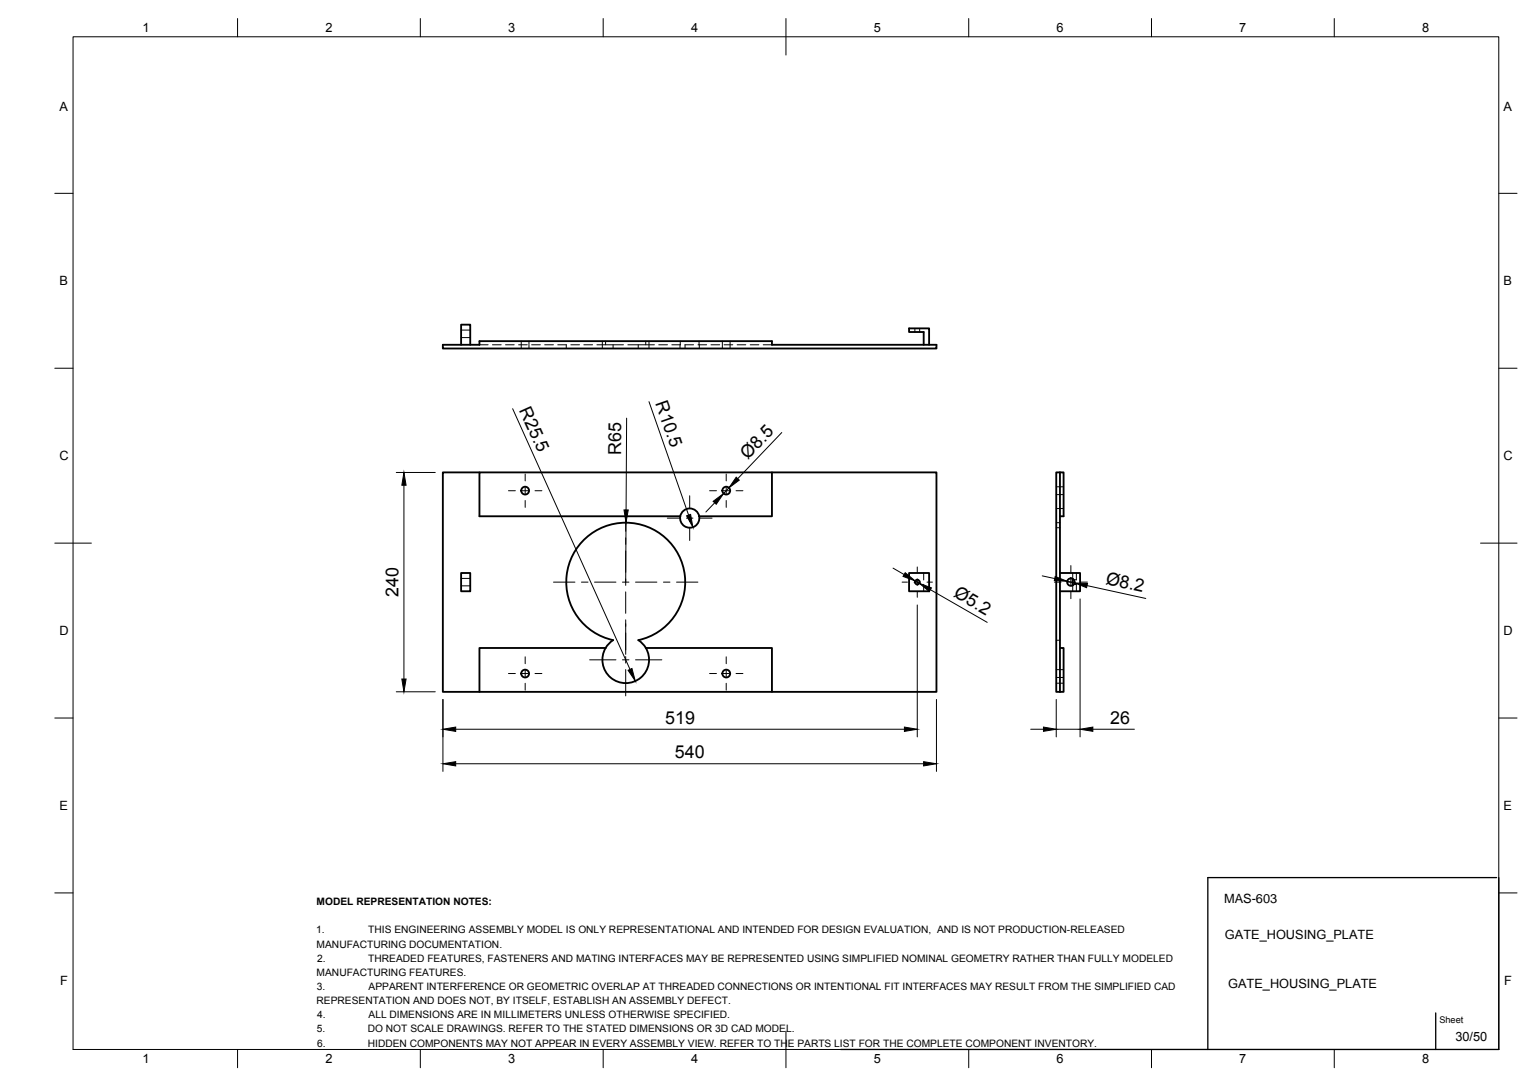
ISO-10303-21;
HEADER;
FILE_DESCRIPTION((''),'2;1');
FILE_NAME('GATE_HOUSING_PLATE.step','2026-10-01T22:06:14-07:00',(''),(''),'','','');
FILE_SCHEMA (('AUTOMOTIVE_DESIGN { 1 0 10303 214 3 1 1 }'));
ENDSEC;
DATA;
#10=MECHANICAL_DESIGN_GEOMETRIC_PRESENTATION_REPRESENTATION('',(#1002),#50440);
#910=SHAPE_REPRESENTATION_RELATIONSHIP('SRR','None',#50643,#955) ;
#955=ADVANCED_BREP_SHAPE_REPRESENTATION('',(#1057),#50412) ;
#1002=STYLED_ITEM('',(#50885),#1057) ;
#1057=MANIFOLD_SOLID_BREP('GATE_HOUSING_PLATE',#28669) ;
#1316=FACE_BOUND('',#5009,.T.) ;
#1317=FACE_BOUND('',#5014,.T.) ;
#1318=FACE_BOUND('',#5021,.T.) ;
#1319=FACE_BOUND('',#5024,.T.) ;
#1320=FACE_BOUND('',#5031,.T.) ;
#1321=FACE_BOUND('',#5032,.T.) ;
#1322=FACE_BOUND('',#5035,.T.) ;
#1323=FACE_BOUND('',#5036,.T.) ;
#1324=FACE_BOUND('',#5042,.T.) ;
#1325=FACE_BOUND('',#5043,.T.) ;
#1326=FACE_BOUND('',#5049,.T.) ;
#1327=FACE_BOUND('',#5050,.T.) ;
#1328=FACE_BOUND('',#5051,.T.) ;
#1329=FACE_BOUND('',#5052,.T.) ;
#1330=FACE_BOUND('',#5053,.T.) ;
#1331=FACE_BOUND('',#5054,.T.) ;
#2103=PLANE('',#30678) ;
#2104=PLANE('',#30679) ;
#2105=PLANE('',#30680) ;
#2106=PLANE('',#30681) ;
#2107=PLANE('',#30682) ;
#2108=PLANE('',#30683) ;
#2109=PLANE('',#30684) ;
#2110=PLANE('',#30688) ;
#2111=PLANE('',#30689) ;
#2112=PLANE('',#30690) ;
#2113=PLANE('',#30691) ;
#2114=PLANE('',#30692) ;
#2115=PLANE('',#30710) ;
#2116=PLANE('',#30714) ;
#2117=PLANE('',#30715) ;
#2118=PLANE('',#30717) ;
#2119=PLANE('',#30718) ;
#2120=PLANE('',#30719) ;
#2121=PLANE('',#30720) ;
#2122=PLANE('',#30721) ;
#2123=PLANE('',#30722) ;
#2124=PLANE('',#30723) ;
#2125=PLANE('',#30724) ;
#2126=PLANE('',#30727) ;
#2127=PLANE('',#30730) ;
#2128=PLANE('',#30731) ;
#2129=PLANE('',#30732) ;
#2130=PLANE('',#30733) ;
#3249=FACE_OUTER_BOUND('',#5007,.T.) ;
#3250=FACE_OUTER_BOUND('',#5008,.T.) ;
#3251=FACE_OUTER_BOUND('',#5010,.T.) ;
#3252=FACE_OUTER_BOUND('',#5011,.T.) ;
#3253=FACE_OUTER_BOUND('',#5012,.T.) ;
#3254=FACE_OUTER_BOUND('',#5013,.T.) ;
#3255=FACE_OUTER_BOUND('',#5015,.T.) ;
#3256=FACE_OUTER_BOUND('',#5016,.T.) ;
#3257=FACE_OUTER_BOUND('',#5017,.T.) ;
#3258=FACE_OUTER_BOUND('',#5018,.T.) ;
#3259=FACE_OUTER_BOUND('',#5019,.T.) ;
#3260=FACE_OUTER_BOUND('',#5020,.T.) ;
#3261=FACE_OUTER_BOUND('',#5022,.T.) ;
#3262=FACE_OUTER_BOUND('',#5023,.T.) ;
#3263=FACE_OUTER_BOUND('',#5025,.T.) ;
#3264=FACE_OUTER_BOUND('',#5026,.T.) ;
#3265=FACE_OUTER_BOUND('',#5027,.T.) ;
#3266=FACE_OUTER_BOUND('',#5028,.T.) ;
#3267=FACE_OUTER_BOUND('',#5029,.T.) ;
#3268=FACE_OUTER_BOUND('',#5030,.T.) ;
#3269=FACE_OUTER_BOUND('',#5033,.T.) ;
#3270=FACE_OUTER_BOUND('',#5034,.T.) ;
#3271=FACE_OUTER_BOUND('',#5037,.T.) ;
#3272=FACE_OUTER_BOUND('',#5038,.T.) ;
#3273=FACE_OUTER_BOUND('',#5039,.T.) ;
#3274=FACE_OUTER_BOUND('',#5040,.T.) ;
#3275=FACE_OUTER_BOUND('',#5041,.T.) ;
#3276=FACE_OUTER_BOUND('',#5044,.T.) ;
#3277=FACE_OUTER_BOUND('',#5045,.T.) ;
#3278=FACE_OUTER_BOUND('',#5046,.T.) ;
#3279=FACE_OUTER_BOUND('',#5047,.T.) ;
#3280=FACE_OUTER_BOUND('',#5048,.T.) ;
#3281=FACE_OUTER_BOUND('',#5055,.T.) ;
#3282=FACE_OUTER_BOUND('',#5056,.T.) ;
#3283=FACE_OUTER_BOUND('',#5057,.T.) ;
#3284=FACE_OUTER_BOUND('',#5058,.T.) ;
#3285=FACE_OUTER_BOUND('',#5059,.T.) ;
#5007=EDGE_LOOP('',(#23237,#23238,#23239,#23240)) ;
#5008=EDGE_LOOP('',(#23241,#23242,#23243,#23244)) ;
#5009=EDGE_LOOP('',(#23245)) ;
#5010=EDGE_LOOP('',(#23246,#23247,#23248,#23249)) ;
#5011=EDGE_LOOP('',(#23250,#23251,#23252,#23253,#23254,#23255)) ;
#5012=EDGE_LOOP('',(#23256,#23257,#23258,#23259)) ;
#5013=EDGE_LOOP('',(#23260,#23261,#23262,#23263)) ;
#5014=EDGE_LOOP('',(#23264)) ;
#5015=EDGE_LOOP('',(#23265,#23266,#23267,#23268,#23269,#23270)) ;
#5016=EDGE_LOOP('',(#23271,#23272,#23273,#23274)) ;
#5017=EDGE_LOOP('',(#23275,#23276,#23277,#23278)) ;
#5018=EDGE_LOOP('',(#23279,#23280,#23281,#23282)) ;
#5019=EDGE_LOOP('',(#23283,#23284,#23285,#23286)) ;
#5020=EDGE_LOOP('',(#23287,#23288,#23289,#23290)) ;
#5021=EDGE_LOOP('',(#23291)) ;
#5022=EDGE_LOOP('',(#23292,#23293,#23294,#23295)) ;
#5023=EDGE_LOOP('',(#23296,#23297,#23298,#23299)) ;
#5024=EDGE_LOOP('',(#23300)) ;
#5025=EDGE_LOOP('',(#23301,#23302,#23303,#23304)) ;
#5026=EDGE_LOOP('',(#23305,#23306,#23307,#23308)) ;
#5027=EDGE_LOOP('',(#23309,#23310,#23311,#23312)) ;
#5028=EDGE_LOOP('',(#23313,#23314,#23315,#23316)) ;
#5029=EDGE_LOOP('',(#23317,#23318,#23319,#23320,#23321,#23322,#23323,#23324)) ;
#5030=EDGE_LOOP('',(#23325,#23326,#23327,#23328,#23329,#23330,#23331,#23332,
#23333,#23334,#23335,#23336,#23337,#23338,#23339,#23340,#23341,#23342,#23343)) ;
#5031=EDGE_LOOP('',(#23344,#23345,#23346,#23347)) ;
#5032=EDGE_LOOP('',(#23348,#23349,#23350,#23351)) ;
#5033=EDGE_LOOP('',(#23352,#23353,#23354,#23355)) ;
#5034=EDGE_LOOP('',(#23356,#23357,#23358,#23359,#23360,#23361)) ;
#5035=EDGE_LOOP('',(#23362)) ;
#5036=EDGE_LOOP('',(#23363)) ;
#5037=EDGE_LOOP('',(#23364,#23365,#23366,#23367)) ;
#5038=EDGE_LOOP('',(#23368,#23369,#23370,#23371)) ;
#5039=EDGE_LOOP('',(#23372,#23373,#23374,#23375)) ;
#5040=EDGE_LOOP('',(#23376,#23377,#23378,#23379)) ;
#5041=EDGE_LOOP('',(#23380,#23381,#23382,#23383,#23384,#23385)) ;
#5042=EDGE_LOOP('',(#23386)) ;
#5043=EDGE_LOOP('',(#23387)) ;
#5044=EDGE_LOOP('',(#23388,#23389,#23390,#23391)) ;
#5045=EDGE_LOOP('',(#23392,#23393,#23394,#23395)) ;
#5046=EDGE_LOOP('',(#23396,#23397,#23398,#23399)) ;
#5047=EDGE_LOOP('',(#23400,#23401,#23402,#23403,#23404,#23405,#23406,#23407)) ;
#5048=EDGE_LOOP('',(#23408,#23409,#23410,#23411)) ;
#5049=EDGE_LOOP('',(#23412)) ;
#5050=EDGE_LOOP('',(#23413)) ;
#5051=EDGE_LOOP('',(#23414)) ;
#5052=EDGE_LOOP('',(#23415)) ;
#5053=EDGE_LOOP('',(#23416)) ;
#5054=EDGE_LOOP('',(#23417,#23418)) ;
#5055=EDGE_LOOP('',(#23419,#23420,#23421,#23422)) ;
#5056=EDGE_LOOP('',(#23423,#23424,#23425,#23426,#23427,#23428,#23429,#23430)) ;
#5057=EDGE_LOOP('',(#23431,#23432,#23433,#23434)) ;
#5058=EDGE_LOOP('',(#23435,#23436,#23437,#23438,#23439,#23440,#23441,#23442)) ;
#5059=EDGE_LOOP('',(#23443,#23444,#23445,#23446)) ;
#7537=LINE('',#46216,#10009) ;
#7538=LINE('',#46221,#10010) ;
#7539=LINE('',#46223,#10011) ;
#7540=LINE('',#46225,#10012) ;
#7541=LINE('',#46226,#10013) ;
#7542=LINE('',#46229,#10014) ;
#7543=LINE('',#46231,#10015) ;
#7544=LINE('',#46232,#10016) ;
#7545=LINE('',#46236,#10017) ;
#7546=LINE('',#46238,#10018) ;
#7547=LINE('',#46239,#10019) ;
#7548=LINE('',#46240,#10020) ;
#7549=LINE('',#46244,#10021) ;
#7550=LINE('',#46245,#10022) ;
#7551=LINE('',#46246,#10023) ;
#7552=LINE('',#46248,#10024) ;
#7553=LINE('',#46251,#10025) ;
#7554=LINE('',#46252,#10026) ;
#7555=LINE('',#46254,#10027) ;
#7556=LINE('',#46259,#10028) ;
#7557=LINE('',#46264,#10029) ;
#7558=LINE('',#46266,#10030) ;
#7559=LINE('',#46268,#10031) ;
#7560=LINE('',#46269,#10032) ;
#7561=LINE('',#46272,#10033) ;
#7562=LINE('',#46274,#10034) ;
#7563=LINE('',#46275,#10035) ;
#7564=LINE('',#46278,#10036) ;
#7565=LINE('',#46279,#10037) ;
#7566=LINE('',#46282,#10038) ;
#7567=LINE('',#46283,#10039) ;
#7568=LINE('',#46285,#10040) ;
#7569=LINE('',#46290,#10041) ;
#7570=LINE('',#46296,#10042) ;
#7571=LINE('',#46302,#10043) ;
#7572=LINE('',#46308,#10044) ;
#7573=LINE('',#46314,#10045) ;
#7574=LINE('',#46318,#10046) ;
#7575=LINE('',#46322,#10047) ;
#7576=LINE('',#46326,#10048) ;
#7577=LINE('',#46328,#10049) ;
#7578=LINE('',#46330,#10050) ;
#7579=LINE('',#46332,#10051) ;
#7580=LINE('',#46334,#10052) ;
#7581=LINE('',#46336,#10053) ;
#7582=LINE('',#46338,#10054) ;
#7583=LINE('',#46346,#10055) ;
#7584=LINE('',#46348,#10056) ;
#7585=LINE('',#46350,#10057) ;
#7586=LINE('',#46352,#10058) ;
#7587=LINE('',#46354,#10059) ;
#7588=LINE('',#46356,#10060) ;
#7589=LINE('',#46357,#10061) ;
#7590=LINE('',#46360,#10062) ;
#7591=LINE('',#46361,#10063) ;
#7592=LINE('',#46367,#10064) ;
#7593=LINE('',#46369,#10065) ;
#7594=LINE('',#46371,#10066) ;
#7595=LINE('',#46373,#10067) ;
#7596=LINE('',#46374,#10068) ;
#7597=LINE('',#46376,#10069) ;
#7598=LINE('',#46377,#10070) ;
#7599=LINE('',#46379,#10071) ;
#7600=LINE('',#46381,#10072) ;
#7601=LINE('',#46382,#10073) ;
#7602=LINE('',#46384,#10074) ;
#7603=LINE('',#46387,#10075) ;
#7604=LINE('',#46389,#10076) ;
#7605=LINE('',#46391,#10077) ;
#7606=LINE('',#46392,#10078) ;
#7607=LINE('',#46394,#10079) ;
#7608=LINE('',#46396,#10080) ;
#7609=LINE('',#46398,#10081) ;
#7610=LINE('',#46401,#10082) ;
#7611=LINE('',#46404,#10083) ;
#7612=LINE('',#46408,#10084) ;
#7613=LINE('',#46410,#10085) ;
#7614=LINE('',#46412,#10086) ;
#7615=LINE('',#46413,#10087) ;
#7616=LINE('',#46417,#10088) ;
#7617=LINE('',#46418,#10089) ;
#7618=LINE('',#46420,#10090) ;
#7619=LINE('',#46422,#10091) ;
#10009=VECTOR('',#37116,0.26) ;
#10010=VECTOR('',#37121,1.) ;
#10011=VECTOR('',#37122,1.) ;
#10012=VECTOR('',#37123,1.) ;
#10013=VECTOR('',#37124,1.) ;
#10014=VECTOR('',#37127,1.) ;
#10015=VECTOR('',#37128,1.) ;
#10016=VECTOR('',#37129,1.) ;
#10017=VECTOR('',#37132,1.) ;
#10018=VECTOR('',#37133,1.) ;
#10019=VECTOR('',#37134,1.) ;
#10020=VECTOR('',#37135,1.) ;
#10021=VECTOR('',#37138,1.) ;
#10022=VECTOR('',#37139,1.) ;
#10023=VECTOR('',#37140,1.) ;
#10024=VECTOR('',#37143,1.) ;
#10025=VECTOR('',#37146,1.) ;
#10026=VECTOR('',#37147,1.) ;
#10027=VECTOR('',#37150,1.) ;
#10028=VECTOR('',#37155,0.41) ;
#10029=VECTOR('',#37160,1.) ;
#10030=VECTOR('',#37161,1.) ;
#10031=VECTOR('',#37162,1.) ;
#10032=VECTOR('',#37163,1.) ;
#10033=VECTOR('',#37166,1.) ;
#10034=VECTOR('',#37167,1.) ;
#10035=VECTOR('',#37168,1.) ;
#10036=VECTOR('',#37171,1.) ;
#10037=VECTOR('',#37172,1.) ;
#10038=VECTOR('',#37175,1.) ;
#10039=VECTOR('',#37176,1.) ;
#10040=VECTOR('',#37179,1.) ;
#10041=VECTOR('',#37184,0.425) ;
#10042=VECTOR('',#37191,0.425) ;
#10043=VECTOR('',#37198,0.425) ;
#10044=VECTOR('',#37205,0.425) ;
#10045=VECTOR('',#37212,1.05) ;
#10046=VECTOR('',#37215,1.) ;
#10047=VECTOR('',#37218,1.) ;
#10048=VECTOR('',#37223,1.) ;
#10049=VECTOR('',#37224,1.) ;
#10050=VECTOR('',#37225,1.) ;
#10051=VECTOR('',#37226,1.) ;
#10052=VECTOR('',#37227,1.) ;
#10053=VECTOR('',#37228,1.) ;
#10054=VECTOR('',#37229,1.) ;
#10055=VECTOR('',#37236,1.) ;
#10056=VECTOR('',#37237,1.) ;
#10057=VECTOR('',#37238,1.) ;
#10058=VECTOR('',#37239,1.) ;
#10059=VECTOR('',#37240,1.) ;
#10060=VECTOR('',#37241,1.) ;
#10061=VECTOR('',#37242,1.) ;
#10062=VECTOR('',#37245,1.) ;
#10063=VECTOR('',#37246,1.) ;
#10064=VECTOR('',#37251,1.) ;
#10065=VECTOR('',#37252,1.) ;
#10066=VECTOR('',#37253,1.) ;
#10067=VECTOR('',#37254,1.) ;
#10068=VECTOR('',#37255,1.) ;
#10069=VECTOR('',#37258,1.) ;
#10070=VECTOR('',#37259,1.) ;
#10071=VECTOR('',#37262,1.) ;
#10072=VECTOR('',#37265,1.) ;
#10073=VECTOR('',#37266,1.) ;
#10074=VECTOR('',#37269,1.) ;
#10075=VECTOR('',#37272,1.) ;
#10076=VECTOR('',#37273,1.) ;
#10077=VECTOR('',#37274,1.) ;
#10078=VECTOR('',#37275,1.) ;
#10079=VECTOR('',#37278,1.) ;
#10080=VECTOR('',#37281,1.) ;
#10081=VECTOR('',#37284,1.) ;
#10082=VECTOR('',#37287,1.) ;
#10083=VECTOR('',#37290,1.) ;
#10084=VECTOR('',#37293,1.) ;
#10085=VECTOR('',#37294,1.) ;
#10086=VECTOR('',#37295,1.) ;
#10087=VECTOR('',#37296,1.) ;
#10088=VECTOR('',#37303,1.) ;
#10089=VECTOR('',#37304,1.) ;
#10090=VECTOR('',#37307,1.) ;
#10091=VECTOR('',#37310,1.) ;
#11151=CIRCLE('',#30676,0.26) ;
#11152=CIRCLE('',#30677,0.26) ;
#11153=CIRCLE('',#30686,0.41) ;
#11154=CIRCLE('',#30687,0.41) ;
#11155=CIRCLE('',#30694,0.425) ;
#11156=CIRCLE('',#30695,0.425) ;
#11157=CIRCLE('',#30697,0.425) ;
#11158=CIRCLE('',#30698,0.425) ;
#11159=CIRCLE('',#30700,0.425) ;
#11160=CIRCLE('',#30701,0.425) ;
#11161=CIRCLE('',#30703,0.425) ;
#11162=CIRCLE('',#30704,0.425) ;
#11163=CIRCLE('',#30706,1.05) ;
#11164=CIRCLE('',#30707,1.05) ;
#11165=CIRCLE('',#30708,1.05) ;
#11166=CIRCLE('',#30709,1.05) ;
#11167=CIRCLE('',#30711,2.55) ;
#11168=CIRCLE('',#30712,6.5) ;
#11169=CIRCLE('',#30713,2.55) ;
#11170=CIRCLE('',#30716,2.55) ;
#11171=CIRCLE('',#30726,2.55) ;
#11172=CIRCLE('',#30728,6.5) ;
#13395=VERTEX_POINT('',#46213) ;
#13396=VERTEX_POINT('',#46215) ;
#13397=VERTEX_POINT('',#46219) ;
#13398=VERTEX_POINT('',#46220) ;
#13399=VERTEX_POINT('',#46222) ;
#13400=VERTEX_POINT('',#46224) ;
#13401=VERTEX_POINT('',#46228) ;
#13402=VERTEX_POINT('',#46230) ;
#13403=VERTEX_POINT('',#46234) ;
#13404=VERTEX_POINT('',#46235) ;
#13405=VERTEX_POINT('',#46237) ;
#13406=VERTEX_POINT('',#46242) ;
#13407=VERTEX_POINT('',#46243) ;
#13408=VERTEX_POINT('',#46250) ;
#13409=VERTEX_POINT('',#46256) ;
#13410=VERTEX_POINT('',#46258) ;
#13411=VERTEX_POINT('',#46262) ;
#13412=VERTEX_POINT('',#46263) ;
#13413=VERTEX_POINT('',#46265) ;
#13414=VERTEX_POINT('',#46267) ;
#13415=VERTEX_POINT('',#46271) ;
#13416=VERTEX_POINT('',#46273) ;
#13417=VERTEX_POINT('',#46277) ;
#13418=VERTEX_POINT('',#46281) ;
#13419=VERTEX_POINT('',#46287) ;
#13420=VERTEX_POINT('',#46289) ;
#13421=VERTEX_POINT('',#46293) ;
#13422=VERTEX_POINT('',#46295) ;
#13423=VERTEX_POINT('',#46299) ;
#13424=VERTEX_POINT('',#46301) ;
#13425=VERTEX_POINT('',#46305) ;
#13426=VERTEX_POINT('',#46307) ;
#13427=VERTEX_POINT('',#46311) ;
#13428=VERTEX_POINT('',#46313) ;
#13429=VERTEX_POINT('',#46315) ;
#13430=VERTEX_POINT('',#46317) ;
#13431=VERTEX_POINT('',#46319) ;
#13432=VERTEX_POINT('',#46321) ;
#13433=VERTEX_POINT('',#46325) ;
#13434=VERTEX_POINT('',#46327) ;
#13435=VERTEX_POINT('',#46329) ;
#13436=VERTEX_POINT('',#46331) ;
#13437=VERTEX_POINT('',#46333) ;
#13438=VERTEX_POINT('',#46335) ;
#13439=VERTEX_POINT('',#46337) ;
#13440=VERTEX_POINT('',#46339) ;
#13441=VERTEX_POINT('',#46341) ;
#13442=VERTEX_POINT('',#46343) ;
#13443=VERTEX_POINT('',#46345) ;
#13444=VERTEX_POINT('',#46347) ;
#13445=VERTEX_POINT('',#46349) ;
#13446=VERTEX_POINT('',#46351) ;
#13447=VERTEX_POINT('',#46353) ;
#13448=VERTEX_POINT('',#46355) ;
#13449=VERTEX_POINT('',#46359) ;
#13450=VERTEX_POINT('',#46363) ;
#13451=VERTEX_POINT('',#46364) ;
#13452=VERTEX_POINT('',#46366) ;
#13453=VERTEX_POINT('',#46368) ;
#13454=VERTEX_POINT('',#46370) ;
#13455=VERTEX_POINT('',#46372) ;
#13456=VERTEX_POINT('',#46386) ;
#13457=VERTEX_POINT('',#46388) ;
#13458=VERTEX_POINT('',#46390) ;
#13459=VERTEX_POINT('',#46400) ;
#13460=VERTEX_POINT('',#46402) ;
#13461=VERTEX_POINT('',#46406) ;
#13462=VERTEX_POINT('',#46407) ;
#13463=VERTEX_POINT('',#46409) ;
#13464=VERTEX_POINT('',#46411) ;
#16884=EDGE_CURVE('',#13395,#13395,#11151,.T.) ;
#16885=EDGE_CURVE('',#13395,#13396,#7537,.T.) ;
#16886=EDGE_CURVE('',#13396,#13396,#11152,.T.) ;
#16887=EDGE_CURVE('',#13397,#13398,#7538,.T.) ;
#16888=EDGE_CURVE('',#13397,#13399,#7539,.T.) ;
#16889=EDGE_CURVE('',#13399,#13400,#7540,.T.) ;
#16890=EDGE_CURVE('',#13400,#13398,#7541,.T.) ;
#16891=EDGE_CURVE('',#13401,#13400,#7542,.T.) ;
#16892=EDGE_CURVE('',#13402,#13399,#7543,.T.) ;
#16893=EDGE_CURVE('',#13401,#13402,#7544,.T.) ;
#16894=EDGE_CURVE('',#13403,#13404,#7545,.T.) ;
#16895=EDGE_CURVE('',#13405,#13404,#7546,.T.) ;
#16896=EDGE_CURVE('',#13398,#13405,#7547,.T.) ;
#16897=EDGE_CURVE('',#13403,#13401,#7548,.T.) ;
#16898=EDGE_CURVE('',#13406,#13407,#7549,.T.) ;
#16899=EDGE_CURVE('',#13404,#13407,#7550,.T.) ;
#16900=EDGE_CURVE('',#13406,#13403,#7551,.T.) ;
#16901=EDGE_CURVE('',#13402,#13406,#7552,.T.) ;
#16902=EDGE_CURVE('',#13397,#13408,#7553,.T.) ;
#16903=EDGE_CURVE('',#13407,#13408,#7554,.T.) ;
#16904=EDGE_CURVE('',#13408,#13405,#7555,.T.) ;
#16905=EDGE_CURVE('',#13409,#13409,#11153,.T.) ;
#16906=EDGE_CURVE('',#13409,#13410,#7556,.T.) ;
#16907=EDGE_CURVE('',#13410,#13410,#11154,.T.) ;
#16908=EDGE_CURVE('',#13411,#13412,#7557,.T.) ;
#16909=EDGE_CURVE('',#13412,#13413,#7558,.T.) ;
#16910=EDGE_CURVE('',#13413,#13414,#7559,.T.) ;
#16911=EDGE_CURVE('',#13414,#13411,#7560,.T.) ;
#16912=EDGE_CURVE('',#13414,#13415,#7561,.T.) ;
#16913=EDGE_CURVE('',#13416,#13415,#7562,.T.) ;
#16914=EDGE_CURVE('',#13411,#13416,#7563,.T.) ;
#16915=EDGE_CURVE('',#13413,#13417,#7564,.T.) ;
#16916=EDGE_CURVE('',#13415,#13417,#7565,.T.) ;
#16917=EDGE_CURVE('',#13412,#13418,#7566,.T.) ;
#16918=EDGE_CURVE('',#13417,#13418,#7567,.T.) ;
#16919=EDGE_CURVE('',#13418,#13416,#7568,.T.) ;
#16920=EDGE_CURVE('',#13419,#13419,#11155,.T.) ;
#16921=EDGE_CURVE('',#13419,#13420,#7569,.T.) ;
#16922=EDGE_CURVE('',#13420,#13420,#11156,.T.) ;
#16923=EDGE_CURVE('',#13421,#13421,#11157,.T.) ;
#16924=EDGE_CURVE('',#13421,#13422,#7570,.T.) ;
#16925=EDGE_CURVE('',#13422,#13422,#11158,.T.) ;
#16926=EDGE_CURVE('',#13423,#13423,#11159,.T.) ;
#16927=EDGE_CURVE('',#13423,#13424,#7571,.T.) ;
#16928=EDGE_CURVE('',#13424,#13424,#11160,.T.) ;
#16929=EDGE_CURVE('',#13425,#13425,#11161,.T.) ;
#16930=EDGE_CURVE('',#13425,#13426,#7572,.T.) ;
#16931=EDGE_CURVE('',#13426,#13426,#11162,.T.) ;
#16932=EDGE_CURVE('',#13427,#13427,#11163,.T.) ;
#16933=EDGE_CURVE('',#13427,#13428,#7573,.T.) ;
#16934=EDGE_CURVE('',#13429,#13428,#11164,.T.) ;
#16935=EDGE_CURVE('',#13430,#13429,#7574,.T.) ;
#16936=EDGE_CURVE('',#13431,#13430,#11165,.T.) ;
#16937=EDGE_CURVE('',#13432,#13431,#7575,.T.) ;
#16938=EDGE_CURVE('',#13428,#13432,#11166,.T.) ;
#16939=EDGE_CURVE('',#13432,#13433,#7576,.T.) ;
#16940=EDGE_CURVE('',#13433,#13434,#7577,.T.) ;
#16941=EDGE_CURVE('',#13434,#13435,#7578,.T.) ;
#16942=EDGE_CURVE('',#13435,#13436,#7579,.T.) ;
#16943=EDGE_CURVE('',#13436,#13437,#7580,.T.) ;
#16944=EDGE_CURVE('',#13437,#13438,#7581,.T.) ;
#16945=EDGE_CURVE('',#13438,#13439,#7582,.T.) ;
#16946=EDGE_CURVE('',#13439,#13440,#11167,.T.) ;
#16947=EDGE_CURVE('',#13440,#13441,#11168,.T.) ;
#16948=EDGE_CURVE('',#13441,#13442,#11169,.T.) ;
#16949=EDGE_CURVE('',#13442,#13443,#7583,.T.) ;
#16950=EDGE_CURVE('',#13443,#13444,#7584,.T.) ;
#16951=EDGE_CURVE('',#13444,#13445,#7585,.T.) ;
#16952=EDGE_CURVE('',#13445,#13446,#7586,.T.) ;
#16953=EDGE_CURVE('',#13446,#13447,#7587,.T.) ;
#16954=EDGE_CURVE('',#13447,#13448,#7588,.T.) ;
#16955=EDGE_CURVE('',#13448,#13429,#7589,.T.) ;
#16956=EDGE_CURVE('',#13449,#13431,#7590,.T.) ;
#16957=EDGE_CURVE('',#13449,#13433,#7591,.T.) ;
#16958=EDGE_CURVE('',#13450,#13451,#11170,.T.) ;
#16959=EDGE_CURVE('',#13451,#13452,#7592,.T.) ;
#16960=EDGE_CURVE('',#13452,#13453,#7593,.T.) ;
#16961=EDGE_CURVE('',#13453,#13454,#7594,.T.) ;
#16962=EDGE_CURVE('',#13454,#13455,#7595,.T.) ;
#16963=EDGE_CURVE('',#13455,#13450,#7596,.T.) ;
#16964=EDGE_CURVE('',#13451,#13439,#7597,.T.) ;
#16965=EDGE_CURVE('',#13452,#13438,#7598,.T.) ;
#16966=EDGE_CURVE('',#13453,#13437,#7599,.T.) ;
#16967=EDGE_CURVE('',#13442,#13450,#7600,.T.) ;
#16968=EDGE_CURVE('',#13455,#13443,#7601,.T.) ;
#16969=EDGE_CURVE('',#13454,#13444,#7602,.T.) ;
#16970=EDGE_CURVE('',#13430,#13456,#7603,.T.) ;
#16971=EDGE_CURVE('',#13456,#13457,#7604,.T.) ;
#16972=EDGE_CURVE('',#13457,#13458,#7605,.T.) ;
#16973=EDGE_CURVE('',#13458,#13449,#7606,.T.) ;
#16974=EDGE_CURVE('',#13456,#13448,#7607,.T.) ;
#16975=EDGE_CURVE('',#13458,#13434,#7608,.T.) ;
#16976=EDGE_CURVE('',#13457,#13447,#7609,.T.) ;
#16977=EDGE_CURVE('',#13459,#13441,#7610,.T.) ;
#16978=EDGE_CURVE('',#13460,#13459,#11171,.T.) ;
#16979=EDGE_CURVE('',#13440,#13460,#7611,.T.) ;
#16980=EDGE_CURVE('',#13461,#13462,#7612,.T.) ;
#16981=EDGE_CURVE('',#13462,#13463,#7613,.T.) ;
#16982=EDGE_CURVE('',#13463,#13464,#7614,.T.) ;
#16983=EDGE_CURVE('',#13464,#13461,#7615,.T.) ;
#16984=EDGE_CURVE('',#13459,#13460,#11172,.T.) ;
#16985=EDGE_CURVE('',#13436,#13463,#7616,.T.) ;
#16986=EDGE_CURVE('',#13445,#13462,#7617,.T.) ;
#16987=EDGE_CURVE('',#13435,#13464,#7618,.T.) ;
#16988=EDGE_CURVE('',#13446,#13461,#7619,.T.) ;
#23237=ORIENTED_EDGE('',*,*,#16884,.F.) ;
#23238=ORIENTED_EDGE('',*,*,#16885,.T.) ;
#23239=ORIENTED_EDGE('',*,*,#16886,.F.) ;
#23240=ORIENTED_EDGE('',*,*,#16885,.F.) ;
#23241=ORIENTED_EDGE('',*,*,#16887,.F.) ;
#23242=ORIENTED_EDGE('',*,*,#16888,.T.) ;
#23243=ORIENTED_EDGE('',*,*,#16889,.T.) ;
#23244=ORIENTED_EDGE('',*,*,#16890,.T.) ;
#23245=ORIENTED_EDGE('',*,*,#16884,.T.) ;
#23246=ORIENTED_EDGE('',*,*,#16891,.T.) ;
#23247=ORIENTED_EDGE('',*,*,#16889,.F.) ;
#23248=ORIENTED_EDGE('',*,*,#16892,.F.) ;
#23249=ORIENTED_EDGE('',*,*,#16893,.F.) ;
#23250=ORIENTED_EDGE('',*,*,#16894,.T.) ;
#23251=ORIENTED_EDGE('',*,*,#16895,.F.) ;
#23252=ORIENTED_EDGE('',*,*,#16896,.F.) ;
#23253=ORIENTED_EDGE('',*,*,#16890,.F.) ;
#23254=ORIENTED_EDGE('',*,*,#16891,.F.) ;
#23255=ORIENTED_EDGE('',*,*,#16897,.F.) ;
#23256=ORIENTED_EDGE('',*,*,#16898,.T.) ;
#23257=ORIENTED_EDGE('',*,*,#16899,.F.) ;
#23258=ORIENTED_EDGE('',*,*,#16894,.F.) ;
#23259=ORIENTED_EDGE('',*,*,#16900,.F.) ;
#23260=ORIENTED_EDGE('',*,*,#16900,.T.) ;
#23261=ORIENTED_EDGE('',*,*,#16897,.T.) ;
#23262=ORIENTED_EDGE('',*,*,#16893,.T.) ;
#23263=ORIENTED_EDGE('',*,*,#16901,.T.) ;
#23264=ORIENTED_EDGE('',*,*,#16886,.T.) ;
#23265=ORIENTED_EDGE('',*,*,#16902,.T.) ;
#23266=ORIENTED_EDGE('',*,*,#16903,.F.) ;
#23267=ORIENTED_EDGE('',*,*,#16898,.F.) ;
#23268=ORIENTED_EDGE('',*,*,#16901,.F.) ;
#23269=ORIENTED_EDGE('',*,*,#16892,.T.) ;
#23270=ORIENTED_EDGE('',*,*,#16888,.F.) ;
#23271=ORIENTED_EDGE('',*,*,#16887,.T.) ;
#23272=ORIENTED_EDGE('',*,*,#16896,.T.) ;
#23273=ORIENTED_EDGE('',*,*,#16904,.F.) ;
#23274=ORIENTED_EDGE('',*,*,#16902,.F.) ;
#23275=ORIENTED_EDGE('',*,*,#16905,.F.) ;
#23276=ORIENTED_EDGE('',*,*,#16906,.T.) ;
#23277=ORIENTED_EDGE('',*,*,#16907,.F.) ;
#23278=ORIENTED_EDGE('',*,*,#16906,.F.) ;
#23279=ORIENTED_EDGE('',*,*,#16908,.T.) ;
#23280=ORIENTED_EDGE('',*,*,#16909,.T.) ;
#23281=ORIENTED_EDGE('',*,*,#16910,.T.) ;
#23282=ORIENTED_EDGE('',*,*,#16911,.T.) ;
#23283=ORIENTED_EDGE('',*,*,#16912,.T.) ;
#23284=ORIENTED_EDGE('',*,*,#16913,.F.) ;
#23285=ORIENTED_EDGE('',*,*,#16914,.F.) ;
#23286=ORIENTED_EDGE('',*,*,#16911,.F.) ;
#23287=ORIENTED_EDGE('',*,*,#16915,.T.) ;
#23288=ORIENTED_EDGE('',*,*,#16916,.F.) ;
#23289=ORIENTED_EDGE('',*,*,#16912,.F.) ;
#23290=ORIENTED_EDGE('',*,*,#16910,.F.) ;
#23291=ORIENTED_EDGE('',*,*,#16905,.T.) ;
#23292=ORIENTED_EDGE('',*,*,#16917,.T.) ;
#23293=ORIENTED_EDGE('',*,*,#16918,.F.) ;
#23294=ORIENTED_EDGE('',*,*,#16915,.F.) ;
#23295=ORIENTED_EDGE('',*,*,#16909,.F.) ;
#23296=ORIENTED_EDGE('',*,*,#16914,.T.) ;
#23297=ORIENTED_EDGE('',*,*,#16919,.F.) ;
#23298=ORIENTED_EDGE('',*,*,#16917,.F.) ;
#23299=ORIENTED_EDGE('',*,*,#16908,.F.) ;
#23300=ORIENTED_EDGE('',*,*,#16907,.T.) ;
#23301=ORIENTED_EDGE('',*,*,#16920,.F.) ;
#23302=ORIENTED_EDGE('',*,*,#16921,.T.) ;
#23303=ORIENTED_EDGE('',*,*,#16922,.F.) ;
#23304=ORIENTED_EDGE('',*,*,#16921,.F.) ;
#23305=ORIENTED_EDGE('',*,*,#16923,.F.) ;
#23306=ORIENTED_EDGE('',*,*,#16924,.T.) ;
#23307=ORIENTED_EDGE('',*,*,#16925,.F.) ;
#23308=ORIENTED_EDGE('',*,*,#16924,.F.) ;
#23309=ORIENTED_EDGE('',*,*,#16926,.F.) ;
#23310=ORIENTED_EDGE('',*,*,#16927,.T.) ;
#23311=ORIENTED_EDGE('',*,*,#16928,.F.) ;
#23312=ORIENTED_EDGE('',*,*,#16927,.F.) ;
#23313=ORIENTED_EDGE('',*,*,#16929,.F.) ;
#23314=ORIENTED_EDGE('',*,*,#16930,.T.) ;
#23315=ORIENTED_EDGE('',*,*,#16931,.F.) ;
#23316=ORIENTED_EDGE('',*,*,#16930,.F.) ;
#23317=ORIENTED_EDGE('',*,*,#16932,.F.) ;
#23318=ORIENTED_EDGE('',*,*,#16933,.T.) ;
#23319=ORIENTED_EDGE('',*,*,#16934,.F.) ;
#23320=ORIENTED_EDGE('',*,*,#16935,.F.) ;
#23321=ORIENTED_EDGE('',*,*,#16936,.F.) ;
#23322=ORIENTED_EDGE('',*,*,#16937,.F.) ;
#23323=ORIENTED_EDGE('',*,*,#16938,.F.) ;
#23324=ORIENTED_EDGE('',*,*,#16933,.F.) ;
#23325=ORIENTED_EDGE('',*,*,#16934,.T.) ;
#23326=ORIENTED_EDGE('',*,*,#16938,.T.) ;
#23327=ORIENTED_EDGE('',*,*,#16939,.T.) ;
#23328=ORIENTED_EDGE('',*,*,#16940,.T.) ;
#23329=ORIENTED_EDGE('',*,*,#16941,.T.) ;
#23330=ORIENTED_EDGE('',*,*,#16942,.T.) ;
#23331=ORIENTED_EDGE('',*,*,#16943,.T.) ;
#23332=ORIENTED_EDGE('',*,*,#16944,.T.) ;
#23333=ORIENTED_EDGE('',*,*,#16945,.T.) ;
#23334=ORIENTED_EDGE('',*,*,#16946,.T.) ;
#23335=ORIENTED_EDGE('',*,*,#16947,.T.) ;
#23336=ORIENTED_EDGE('',*,*,#16948,.T.) ;
#23337=ORIENTED_EDGE('',*,*,#16949,.T.) ;
#23338=ORIENTED_EDGE('',*,*,#16950,.T.) ;
#23339=ORIENTED_EDGE('',*,*,#16951,.T.) ;
#23340=ORIENTED_EDGE('',*,*,#16952,.T.) ;
#23341=ORIENTED_EDGE('',*,*,#16953,.T.) ;
#23342=ORIENTED_EDGE('',*,*,#16954,.T.) ;
#23343=ORIENTED_EDGE('',*,*,#16955,.T.) ;
#23344=ORIENTED_EDGE('',*,*,#16903,.T.) ;
#23345=ORIENTED_EDGE('',*,*,#16904,.T.) ;
#23346=ORIENTED_EDGE('',*,*,#16895,.T.) ;
#23347=ORIENTED_EDGE('',*,*,#16899,.T.) ;
#23348=ORIENTED_EDGE('',*,*,#16913,.T.) ;
#23349=ORIENTED_EDGE('',*,*,#16916,.T.) ;
#23350=ORIENTED_EDGE('',*,*,#16918,.T.) ;
#23351=ORIENTED_EDGE('',*,*,#16919,.T.) ;
#23352=ORIENTED_EDGE('',*,*,#16937,.T.) ;
#23353=ORIENTED_EDGE('',*,*,#16956,.F.) ;
#23354=ORIENTED_EDGE('',*,*,#16957,.T.) ;
#23355=ORIENTED_EDGE('',*,*,#16939,.F.) ;
#23356=ORIENTED_EDGE('',*,*,#16958,.T.) ;
#23357=ORIENTED_EDGE('',*,*,#16959,.T.) ;
#23358=ORIENTED_EDGE('',*,*,#16960,.T.) ;
#23359=ORIENTED_EDGE('',*,*,#16961,.T.) ;
#23360=ORIENTED_EDGE('',*,*,#16962,.T.) ;
#23361=ORIENTED_EDGE('',*,*,#16963,.T.) ;
#23362=ORIENTED_EDGE('',*,*,#16922,.T.) ;
#23363=ORIENTED_EDGE('',*,*,#16928,.T.) ;
#23364=ORIENTED_EDGE('',*,*,#16964,.T.) ;
#23365=ORIENTED_EDGE('',*,*,#16945,.F.) ;
#23366=ORIENTED_EDGE('',*,*,#16965,.F.) ;
#23367=ORIENTED_EDGE('',*,*,#16959,.F.) ;
#23368=ORIENTED_EDGE('',*,*,#16965,.T.) ;
#23369=ORIENTED_EDGE('',*,*,#16944,.F.) ;
#23370=ORIENTED_EDGE('',*,*,#16966,.F.) ;
#23371=ORIENTED_EDGE('',*,*,#16960,.F.) ;
#23372=ORIENTED_EDGE('',*,*,#16967,.T.) ;
#23373=ORIENTED_EDGE('',*,*,#16963,.F.) ;
#23374=ORIENTED_EDGE('',*,*,#16968,.T.) ;
#23375=ORIENTED_EDGE('',*,*,#16949,.F.) ;
#23376=ORIENTED_EDGE('',*,*,#16969,.T.) ;
#23377=ORIENTED_EDGE('',*,*,#16950,.F.) ;
#23378=ORIENTED_EDGE('',*,*,#16968,.F.) ;
#23379=ORIENTED_EDGE('',*,*,#16962,.F.) ;
#23380=ORIENTED_EDGE('',*,*,#16936,.T.) ;
#23381=ORIENTED_EDGE('',*,*,#16970,.T.) ;
#23382=ORIENTED_EDGE('',*,*,#16971,.T.) ;
#23383=ORIENTED_EDGE('',*,*,#16972,.T.) ;
#23384=ORIENTED_EDGE('',*,*,#16973,.T.) ;
#23385=ORIENTED_EDGE('',*,*,#16956,.T.) ;
#23386=ORIENTED_EDGE('',*,*,#16925,.T.) ;
#23387=ORIENTED_EDGE('',*,*,#16931,.T.) ;
#23388=ORIENTED_EDGE('',*,*,#16935,.T.) ;
#23389=ORIENTED_EDGE('',*,*,#16955,.F.) ;
#23390=ORIENTED_EDGE('',*,*,#16974,.F.) ;
#23391=ORIENTED_EDGE('',*,*,#16970,.F.) ;
#23392=ORIENTED_EDGE('',*,*,#16975,.T.) ;
#23393=ORIENTED_EDGE('',*,*,#16940,.F.) ;
#23394=ORIENTED_EDGE('',*,*,#16957,.F.) ;
#23395=ORIENTED_EDGE('',*,*,#16973,.F.) ;
#23396=ORIENTED_EDGE('',*,*,#16974,.T.) ;
#23397=ORIENTED_EDGE('',*,*,#16954,.F.) ;
#23398=ORIENTED_EDGE('',*,*,#16976,.F.) ;
#23399=ORIENTED_EDGE('',*,*,#16971,.F.) ;
#23400=ORIENTED_EDGE('',*,*,#16977,.F.) ;
#23401=ORIENTED_EDGE('',*,*,#16978,.F.) ;
#23402=ORIENTED_EDGE('',*,*,#16979,.F.) ;
#23403=ORIENTED_EDGE('',*,*,#16946,.F.) ;
#23404=ORIENTED_EDGE('',*,*,#16964,.F.) ;
#23405=ORIENTED_EDGE('',*,*,#16958,.F.) ;
#23406=ORIENTED_EDGE('',*,*,#16967,.F.) ;
#23407=ORIENTED_EDGE('',*,*,#16948,.F.) ;
#23408=ORIENTED_EDGE('',*,*,#16980,.T.) ;
#23409=ORIENTED_EDGE('',*,*,#16981,.T.) ;
#23410=ORIENTED_EDGE('',*,*,#16982,.T.) ;
#23411=ORIENTED_EDGE('',*,*,#16983,.T.) ;
#23412=ORIENTED_EDGE('',*,*,#16920,.T.) ;
#23413=ORIENTED_EDGE('',*,*,#16923,.T.) ;
#23414=ORIENTED_EDGE('',*,*,#16926,.T.) ;
#23415=ORIENTED_EDGE('',*,*,#16929,.T.) ;
#23416=ORIENTED_EDGE('',*,*,#16932,.T.) ;
#23417=ORIENTED_EDGE('',*,*,#16978,.T.) ;
#23418=ORIENTED_EDGE('',*,*,#16984,.T.) ;
#23419=ORIENTED_EDGE('',*,*,#16979,.T.) ;
#23420=ORIENTED_EDGE('',*,*,#16984,.F.) ;
#23421=ORIENTED_EDGE('',*,*,#16977,.T.) ;
#23422=ORIENTED_EDGE('',*,*,#16947,.F.) ;
#23423=ORIENTED_EDGE('',*,*,#16985,.T.) ;
#23424=ORIENTED_EDGE('',*,*,#16981,.F.) ;
#23425=ORIENTED_EDGE('',*,*,#16986,.F.) ;
#23426=ORIENTED_EDGE('',*,*,#16951,.F.) ;
#23427=ORIENTED_EDGE('',*,*,#16969,.F.) ;
#23428=ORIENTED_EDGE('',*,*,#16961,.F.) ;
#23429=ORIENTED_EDGE('',*,*,#16966,.T.) ;
#23430=ORIENTED_EDGE('',*,*,#16943,.F.) ;
#23431=ORIENTED_EDGE('',*,*,#16987,.T.) ;
#23432=ORIENTED_EDGE('',*,*,#16982,.F.) ;
#23433=ORIENTED_EDGE('',*,*,#16985,.F.) ;
#23434=ORIENTED_EDGE('',*,*,#16942,.F.) ;
#23435=ORIENTED_EDGE('',*,*,#16988,.T.) ;
#23436=ORIENTED_EDGE('',*,*,#16983,.F.) ;
#23437=ORIENTED_EDGE('',*,*,#16987,.F.) ;
#23438=ORIENTED_EDGE('',*,*,#16941,.F.) ;
#23439=ORIENTED_EDGE('',*,*,#16975,.F.) ;
#23440=ORIENTED_EDGE('',*,*,#16972,.F.) ;
#23441=ORIENTED_EDGE('',*,*,#16976,.T.) ;
#23442=ORIENTED_EDGE('',*,*,#16953,.F.) ;
#23443=ORIENTED_EDGE('',*,*,#16986,.T.) ;
#23444=ORIENTED_EDGE('',*,*,#16980,.F.) ;
#23445=ORIENTED_EDGE('',*,*,#16988,.F.) ;
#23446=ORIENTED_EDGE('',*,*,#16952,.F.) ;
#26835=CYLINDRICAL_SURFACE('',#30675,0.26) ;
#26836=CYLINDRICAL_SURFACE('',#30685,0.41) ;
#26837=CYLINDRICAL_SURFACE('',#30693,0.425) ;
#26838=CYLINDRICAL_SURFACE('',#30696,0.425) ;
#26839=CYLINDRICAL_SURFACE('',#30699,0.425) ;
#26840=CYLINDRICAL_SURFACE('',#30702,0.425) ;
#26841=CYLINDRICAL_SURFACE('',#30705,1.05) ;
#26842=CYLINDRICAL_SURFACE('',#30725,2.55) ;
#26843=CYLINDRICAL_SURFACE('',#30729,6.5) ;
#27984=ADVANCED_FACE('',(#3249),#26835,.F.) ;
#27985=ADVANCED_FACE('',(#3250,#1316),#2103,.F.) ;
#27986=ADVANCED_FACE('',(#3251),#2104,.F.) ;
#27987=ADVANCED_FACE('',(#3252),#2105,.F.) ;
#27988=ADVANCED_FACE('',(#3253),#2106,.F.) ;
#27989=ADVANCED_FACE('',(#3254,#1317),#2107,.T.) ;
#27990=ADVANCED_FACE('',(#3255),#2108,.F.) ;
#27991=ADVANCED_FACE('',(#3256),#2109,.F.) ;
#27992=ADVANCED_FACE('',(#3257),#26836,.F.) ;
#27993=ADVANCED_FACE('',(#3258),#2110,.T.) ;
#27994=ADVANCED_FACE('',(#3259),#2111,.F.) ;
#27995=ADVANCED_FACE('',(#3260,#1318),#2112,.F.) ;
#27996=ADVANCED_FACE('',(#3261),#2113,.F.) ;
#27997=ADVANCED_FACE('',(#3262,#1319),#2114,.F.) ;
#27998=ADVANCED_FACE('',(#3263),#26837,.F.) ;
#27999=ADVANCED_FACE('',(#3264),#26838,.F.) ;
#28000=ADVANCED_FACE('',(#3265),#26839,.F.) ;
#28001=ADVANCED_FACE('',(#3266),#26840,.F.) ;
#28002=ADVANCED_FACE('',(#3267),#26841,.F.) ;
#28003=ADVANCED_FACE('',(#3268,#1320,#1321),#2115,.T.) ;
#28004=ADVANCED_FACE('',(#3269),#2116,.F.) ;
#28005=ADVANCED_FACE('',(#3270,#1322,#1323),#2117,.T.) ;
#28006=ADVANCED_FACE('',(#3271),#2118,.F.) ;
#28007=ADVANCED_FACE('',(#3272),#2119,.F.) ;
#28008=ADVANCED_FACE('',(#3273),#2120,.F.) ;
#28009=ADVANCED_FACE('',(#3274),#2121,.F.) ;
#28010=ADVANCED_FACE('',(#3275,#1324,#1325),#2122,.T.) ;
#28011=ADVANCED_FACE('',(#3276),#2123,.F.) ;
#28012=ADVANCED_FACE('',(#3277),#2124,.F.) ;
#28013=ADVANCED_FACE('',(#3278),#2125,.F.) ;
#28014=ADVANCED_FACE('',(#3279),#26842,.F.) ;
#28015=ADVANCED_FACE('',(#3280,#1326,#1327,#1328,#1329,#1330,#1331),#2126,
 .F.) ;
#28016=ADVANCED_FACE('',(#3281),#26843,.F.) ;
#28017=ADVANCED_FACE('',(#3282),#2127,.F.) ;
#28018=ADVANCED_FACE('',(#3283),#2128,.F.) ;
#28019=ADVANCED_FACE('',(#3284),#2129,.F.) ;
#28020=ADVANCED_FACE('',(#3285),#2130,.F.) ;
#28669=CLOSED_SHELL('',(#27984,#27985,#27986,#27987,#27988,#27989,#27990,
#27991,#27992,#27993,#27994,#27995,#27996,#27997,#27998,#27999,#28000,#28001,
#28002,#28003,#28004,#28005,#28006,#28007,#28008,#28009,#28010,#28011,#28012,
#28013,#28014,#28015,#28016,#28017,#28018,#28019,#28020)) ;
#30674=AXIS2_PLACEMENT_3D('',#46211,#37110,#37111) ;
#30675=AXIS2_PLACEMENT_3D('',#46212,#37112,#37113) ;
#30676=AXIS2_PLACEMENT_3D('',#46214,#37114,#37115) ;
#30677=AXIS2_PLACEMENT_3D('',#46217,#37117,#37118) ;
#30678=AXIS2_PLACEMENT_3D('',#46218,#37119,#37120) ;
#30679=AXIS2_PLACEMENT_3D('',#46227,#37125,#37126) ;
#30680=AXIS2_PLACEMENT_3D('',#46233,#37130,#37131) ;
#30681=AXIS2_PLACEMENT_3D('',#46241,#37136,#37137) ;
#30682=AXIS2_PLACEMENT_3D('',#46247,#37141,#37142) ;
#30683=AXIS2_PLACEMENT_3D('',#46249,#37144,#37145) ;
#30684=AXIS2_PLACEMENT_3D('',#46253,#37148,#37149) ;
#30685=AXIS2_PLACEMENT_3D('',#46255,#37151,#37152) ;
#30686=AXIS2_PLACEMENT_3D('',#46257,#37153,#37154) ;
#30687=AXIS2_PLACEMENT_3D('',#46260,#37156,#37157) ;
#30688=AXIS2_PLACEMENT_3D('',#46261,#37158,#37159) ;
#30689=AXIS2_PLACEMENT_3D('',#46270,#37164,#37165) ;
#30690=AXIS2_PLACEMENT_3D('',#46276,#37169,#37170) ;
#30691=AXIS2_PLACEMENT_3D('',#46280,#37173,#37174) ;
#30692=AXIS2_PLACEMENT_3D('',#46284,#37177,#37178) ;
#30693=AXIS2_PLACEMENT_3D('',#46286,#37180,#37181) ;
#30694=AXIS2_PLACEMENT_3D('',#46288,#37182,#37183) ;
#30695=AXIS2_PLACEMENT_3D('',#46291,#37185,#37186) ;
#30696=AXIS2_PLACEMENT_3D('',#46292,#37187,#37188) ;
#30697=AXIS2_PLACEMENT_3D('',#46294,#37189,#37190) ;
#30698=AXIS2_PLACEMENT_3D('',#46297,#37192,#37193) ;
#30699=AXIS2_PLACEMENT_3D('',#46298,#37194,#37195) ;
#30700=AXIS2_PLACEMENT_3D('',#46300,#37196,#37197) ;
#30701=AXIS2_PLACEMENT_3D('',#46303,#37199,#37200) ;
#30702=AXIS2_PLACEMENT_3D('',#46304,#37201,#37202) ;
#30703=AXIS2_PLACEMENT_3D('',#46306,#37203,#37204) ;
#30704=AXIS2_PLACEMENT_3D('',#46309,#37206,#37207) ;
#30705=AXIS2_PLACEMENT_3D('',#46310,#37208,#37209) ;
#30706=AXIS2_PLACEMENT_3D('',#46312,#37210,#37211) ;
#30707=AXIS2_PLACEMENT_3D('',#46316,#37213,#37214) ;
#30708=AXIS2_PLACEMENT_3D('',#46320,#37216,#37217) ;
#30709=AXIS2_PLACEMENT_3D('',#46323,#37219,#37220) ;
#30710=AXIS2_PLACEMENT_3D('',#46324,#37221,#37222) ;
#30711=AXIS2_PLACEMENT_3D('',#46340,#37230,#37231) ;
#30712=AXIS2_PLACEMENT_3D('',#46342,#37232,#37233) ;
#30713=AXIS2_PLACEMENT_3D('',#46344,#37234,#37235) ;
#30714=AXIS2_PLACEMENT_3D('',#46358,#37243,#37244) ;
#30715=AXIS2_PLACEMENT_3D('',#46362,#37247,#37248) ;
#30716=AXIS2_PLACEMENT_3D('',#46365,#37249,#37250) ;
#30717=AXIS2_PLACEMENT_3D('',#46375,#37256,#37257) ;
#30718=AXIS2_PLACEMENT_3D('',#46378,#37260,#37261) ;
#30719=AXIS2_PLACEMENT_3D('',#46380,#37263,#37264) ;
#30720=AXIS2_PLACEMENT_3D('',#46383,#37267,#37268) ;
#30721=AXIS2_PLACEMENT_3D('',#46385,#37270,#37271) ;
#30722=AXIS2_PLACEMENT_3D('',#46393,#37276,#37277) ;
#30723=AXIS2_PLACEMENT_3D('',#46395,#37279,#37280) ;
#30724=AXIS2_PLACEMENT_3D('',#46397,#37282,#37283) ;
#30725=AXIS2_PLACEMENT_3D('',#46399,#37285,#37286) ;
#30726=AXIS2_PLACEMENT_3D('',#46403,#37288,#37289) ;
#30727=AXIS2_PLACEMENT_3D('',#46405,#37291,#37292) ;
#30728=AXIS2_PLACEMENT_3D('',#46414,#37297,#37298) ;
#30729=AXIS2_PLACEMENT_3D('',#46415,#37299,#37300) ;
#30730=AXIS2_PLACEMENT_3D('',#46416,#37301,#37302) ;
#30731=AXIS2_PLACEMENT_3D('',#46419,#37305,#37306) ;
#30732=AXIS2_PLACEMENT_3D('',#46421,#37308,#37309) ;
#30733=AXIS2_PLACEMENT_3D('',#46423,#37311,#37312) ;
#37110=DIRECTION('axis',(0.,0.,1.)) ;
#37111=DIRECTION('refdir',(1.,0.,0.)) ;
#37112=DIRECTION('center_axis',(0.,0.,1.)) ;
#37113=DIRECTION('ref_axis',(1.,0.,0.)) ;
#37114=DIRECTION('center_axis',(0.,0.,1.)) ;
#37115=DIRECTION('ref_axis',(1.,0.,0.)) ;
#37116=DIRECTION('',(0.,0.,1.)) ;
#37117=DIRECTION('center_axis',(0.,0.,-1.)) ;
#37118=DIRECTION('ref_axis',(1.,0.,0.)) ;
#37119=DIRECTION('center_axis',(0.,0.,1.)) ;
#37120=DIRECTION('ref_axis',(1.,0.,0.)) ;
#37121=DIRECTION('',(0.,1.,0.)) ;
#37122=DIRECTION('',(-1.,0.,0.)) ;
#37123=DIRECTION('',(0.,1.,0.)) ;
#37124=DIRECTION('',(1.,0.,0.)) ;
#37125=DIRECTION('center_axis',(1.,0.,0.)) ;
#37126=DIRECTION('ref_axis',(0.,0.,-1.)) ;
#37127=DIRECTION('',(0.,0.,-1.)) ;
#37128=DIRECTION('',(0.,0.,-1.)) ;
#37129=DIRECTION('',(0.,-1.,0.)) ;
#37130=DIRECTION('center_axis',(0.,-1.,0.)) ;
#37131=DIRECTION('ref_axis',(0.,0.,-1.)) ;
#37132=DIRECTION('',(0.,0.,-1.)) ;
#37133=DIRECTION('',(1.,0.,0.)) ;
#37134=DIRECTION('',(0.,0.,-1.)) ;
#37135=DIRECTION('',(-1.,0.,0.)) ;
#37136=DIRECTION('center_axis',(-1.,0.,0.)) ;
#37137=DIRECTION('ref_axis',(0.,0.,1.)) ;
#37138=DIRECTION('',(0.,0.,-1.)) ;
#37139=DIRECTION('',(0.,-1.,0.)) ;
#37140=DIRECTION('',(0.,1.,0.)) ;
#37141=DIRECTION('center_axis',(0.,0.,1.)) ;
#37142=DIRECTION('ref_axis',(1.,0.,0.)) ;
#37143=DIRECTION('',(1.,0.,0.)) ;
#37144=DIRECTION('center_axis',(0.,1.,0.)) ;
#37145=DIRECTION('ref_axis',(0.,0.,1.)) ;
#37146=DIRECTION('',(0.,0.,-1.)) ;
#37147=DIRECTION('',(-1.,0.,0.)) ;
#37148=DIRECTION('center_axis',(1.,0.,0.)) ;
#37149=DIRECTION('ref_axis',(0.,0.,-1.)) ;
#37150=DIRECTION('',(0.,1.,0.)) ;
#37151=DIRECTION('center_axis',(1.,0.,0.)) ;
#37152=DIRECTION('ref_axis',(0.,0.,-1.)) ;
#37153=DIRECTION('center_axis',(1.,0.,0.)) ;
#37154=DIRECTION('ref_axis',(0.,0.,-1.)) ;
#37155=DIRECTION('',(1.,0.,0.)) ;
#37156=DIRECTION('center_axis',(-1.,0.,0.)) ;
#37157=DIRECTION('ref_axis',(0.,0.,-1.)) ;
#37158=DIRECTION('center_axis',(0.,0.,1.)) ;
#37159=DIRECTION('ref_axis',(1.,0.,0.)) ;
#37160=DIRECTION('',(0.,1.,0.)) ;
#37161=DIRECTION('',(-1.,0.,0.)) ;
#37162=DIRECTION('',(0.,-1.,0.)) ;
#37163=DIRECTION('',(1.,0.,0.)) ;
#37164=DIRECTION('center_axis',(0.,1.,0.)) ;
#37165=DIRECTION('ref_axis',(0.,0.,1.)) ;
#37166=DIRECTION('',(0.,0.,-1.)) ;
#37167=DIRECTION('',(-1.,0.,0.)) ;
#37168=DIRECTION('',(0.,0.,-1.)) ;
#37169=DIRECTION('center_axis',(1.,0.,0.)) ;
#37170=DIRECTION('ref_axis',(0.,0.,-1.)) ;
#37171=DIRECTION('',(0.,0.,-1.)) ;
#37172=DIRECTION('',(0.,1.,0.)) ;
#37173=DIRECTION('center_axis',(0.,-1.,0.)) ;
#37174=DIRECTION('ref_axis',(0.,0.,-1.)) ;
#37175=DIRECTION('',(0.,0.,-1.)) ;
#37176=DIRECTION('',(1.,0.,0.)) ;
#37177=DIRECTION('center_axis',(-1.,0.,0.)) ;
#37178=DIRECTION('ref_axis',(0.,0.,1.)) ;
#37179=DIRECTION('',(0.,-1.,0.)) ;
#37180=DIRECTION('center_axis',(0.,0.,1.)) ;
#37181=DIRECTION('ref_axis',(1.,0.,0.)) ;
#37182=DIRECTION('center_axis',(0.,0.,1.)) ;
#37183=DIRECTION('ref_axis',(1.,0.,0.)) ;
#37184=DIRECTION('',(0.,0.,1.)) ;
#37185=DIRECTION('center_axis',(0.,0.,-1.)) ;
#37186=DIRECTION('ref_axis',(1.,0.,0.)) ;
#37187=DIRECTION('center_axis',(0.,0.,1.)) ;
#37188=DIRECTION('ref_axis',(1.,0.,0.)) ;
#37189=DIRECTION('center_axis',(0.,0.,1.)) ;
#37190=DIRECTION('ref_axis',(1.,0.,0.)) ;
#37191=DIRECTION('',(0.,0.,1.)) ;
#37192=DIRECTION('center_axis',(0.,0.,-1.)) ;
#37193=DIRECTION('ref_axis',(1.,0.,0.)) ;
#37194=DIRECTION('center_axis',(0.,0.,1.)) ;
#37195=DIRECTION('ref_axis',(1.,0.,0.)) ;
#37196=DIRECTION('center_axis',(0.,0.,1.)) ;
#37197=DIRECTION('ref_axis',(1.,0.,0.)) ;
#37198=DIRECTION('',(0.,0.,1.)) ;
#37199=DIRECTION('center_axis',(0.,0.,-1.)) ;
#37200=DIRECTION('ref_axis',(1.,0.,0.)) ;
#37201=DIRECTION('center_axis',(0.,0.,1.)) ;
#37202=DIRECTION('ref_axis',(1.,0.,0.)) ;
#37203=DIRECTION('center_axis',(0.,0.,1.)) ;
#37204=DIRECTION('ref_axis',(1.,0.,0.)) ;
#37205=DIRECTION('',(0.,0.,1.)) ;
#37206=DIRECTION('center_axis',(0.,0.,-1.)) ;
#37207=DIRECTION('ref_axis',(1.,0.,0.)) ;
#37208=DIRECTION('center_axis',(0.,0.,1.)) ;
#37209=DIRECTION('ref_axis',(1.,0.,0.)) ;
#37210=DIRECTION('center_axis',(0.,0.,1.)) ;
#37211=DIRECTION('ref_axis',(1.,0.,0.)) ;
#37212=DIRECTION('',(0.,0.,1.)) ;
#37213=DIRECTION('center_axis',(0.,0.,-1.)) ;
#37214=DIRECTION('ref_axis',(1.,0.,0.)) ;
#37215=DIRECTION('',(0.,0.,-1.)) ;
#37216=DIRECTION('center_axis',(0.,0.,-1.)) ;
#37217=DIRECTION('ref_axis',(1.,0.,0.)) ;
#37218=DIRECTION('',(0.,0.,1.)) ;
#37219=DIRECTION('center_axis',(0.,0.,-1.)) ;
#37220=DIRECTION('ref_axis',(1.,0.,0.)) ;
#37221=DIRECTION('center_axis',(0.,0.,1.)) ;
#37222=DIRECTION('ref_axis',(1.,0.,0.)) ;
#37223=DIRECTION('',(-1.,0.,0.)) ;
#37224=DIRECTION('',(0.,1.,0.)) ;
#37225=DIRECTION('',(-1.,0.,0.)) ;
#37226=DIRECTION('',(0.,-1.,0.)) ;
#37227=DIRECTION('',(1.,0.,0.)) ;
#37228=DIRECTION('',(0.,1.,0.)) ;
#37229=DIRECTION('',(1.,0.,0.)) ;
#37230=DIRECTION('center_axis',(0.,0.,-1.)) ;
#37231=DIRECTION('ref_axis',(1.,0.,0.)) ;
#37232=DIRECTION('center_axis',(0.,0.,-1.)) ;
#37233=DIRECTION('ref_axis',(1.,0.,0.)) ;
#37234=DIRECTION('center_axis',(0.,0.,-1.)) ;
#37235=DIRECTION('ref_axis',(1.,0.,0.)) ;
#37236=DIRECTION('',(1.,0.,0.)) ;
#37237=DIRECTION('',(0.,-1.,0.)) ;
#37238=DIRECTION('',(1.,0.,0.)) ;
#37239=DIRECTION('',(0.,1.,0.)) ;
#37240=DIRECTION('',(-1.,0.,0.)) ;
#37241=DIRECTION('',(0.,-1.,0.)) ;
#37242=DIRECTION('',(-1.,0.,0.)) ;
#37243=DIRECTION('center_axis',(0.,1.,0.)) ;
#37244=DIRECTION('ref_axis',(0.,0.,1.)) ;
#37245=DIRECTION('',(1.,0.,0.)) ;
#37246=DIRECTION('',(0.,0.,-1.)) ;
#37247=DIRECTION('center_axis',(0.,0.,1.)) ;
#37248=DIRECTION('ref_axis',(1.,0.,0.)) ;
#37249=DIRECTION('center_axis',(0.,0.,-1.)) ;
#37250=DIRECTION('ref_axis',(1.,0.,0.)) ;
#37251=DIRECTION('',(-1.,0.,0.)) ;
#37252=DIRECTION('',(0.,-1.,0.)) ;
#37253=DIRECTION('',(1.,0.,0.)) ;
#37254=DIRECTION('',(0.,1.,0.)) ;
#37255=DIRECTION('',(-1.,0.,0.)) ;
#37256=DIRECTION('center_axis',(0.,-1.,0.)) ;
#37257=DIRECTION('ref_axis',(0.,0.,-1.)) ;
#37258=DIRECTION('',(0.,0.,-1.)) ;
#37259=DIRECTION('',(0.,0.,-1.)) ;
#37260=DIRECTION('center_axis',(1.,0.,0.)) ;
#37261=DIRECTION('ref_axis',(0.,0.,-1.)) ;
#37262=DIRECTION('',(0.,0.,-1.)) ;
#37263=DIRECTION('center_axis',(0.,-1.,0.)) ;
#37264=DIRECTION('ref_axis',(0.,0.,-1.)) ;
#37265=DIRECTION('',(0.,0.,1.)) ;
#37266=DIRECTION('',(0.,0.,-1.)) ;
#37267=DIRECTION('center_axis',(-1.,0.,0.)) ;
#37268=DIRECTION('ref_axis',(0.,0.,1.)) ;
#37269=DIRECTION('',(0.,0.,-1.)) ;
#37270=DIRECTION('center_axis',(0.,0.,1.)) ;
#37271=DIRECTION('ref_axis',(1.,0.,0.)) ;
#37272=DIRECTION('',(1.,0.,0.)) ;
#37273=DIRECTION('',(0.,1.,0.)) ;
#37274=DIRECTION('',(-1.,0.,0.)) ;
#37275=DIRECTION('',(0.,-1.,0.)) ;
#37276=DIRECTION('center_axis',(0.,1.,0.)) ;
#37277=DIRECTION('ref_axis',(0.,0.,1.)) ;
#37278=DIRECTION('',(0.,0.,-1.)) ;
#37279=DIRECTION('center_axis',(1.,0.,0.)) ;
#37280=DIRECTION('ref_axis',(0.,0.,-1.)) ;
#37281=DIRECTION('',(0.,0.,-1.)) ;
#37282=DIRECTION('center_axis',(-1.,0.,0.)) ;
#37283=DIRECTION('ref_axis',(0.,0.,1.)) ;
#37284=DIRECTION('',(0.,0.,-1.)) ;
#37285=DIRECTION('center_axis',(0.,0.,1.)) ;
#37286=DIRECTION('ref_axis',(6.12323399573677E-17,-1.,0.)) ;
#37287=DIRECTION('',(0.,0.,1.)) ;
#37288=DIRECTION('center_axis',(0.,0.,1.)) ;
#37289=DIRECTION('ref_axis',(1.,0.,0.)) ;
#37290=DIRECTION('',(0.,0.,-1.)) ;
#37291=DIRECTION('center_axis',(0.,0.,1.)) ;
#37292=DIRECTION('ref_axis',(1.,0.,0.)) ;
#37293=DIRECTION('',(0.,-1.,0.)) ;
#37294=DIRECTION('',(-1.,0.,0.)) ;
#37295=DIRECTION('',(0.,1.,0.)) ;
#37296=DIRECTION('',(1.,0.,0.)) ;
#37297=DIRECTION('center_axis',(0.,0.,1.)) ;
#37298=DIRECTION('ref_axis',(1.,0.,0.)) ;
#37299=DIRECTION('center_axis',(0.,0.,1.)) ;
#37300=DIRECTION('ref_axis',(-1.83697019872103E-16,1.,0.)) ;
#37301=DIRECTION('center_axis',(0.,1.,0.)) ;
#37302=DIRECTION('ref_axis',(0.,0.,1.)) ;
#37303=DIRECTION('',(0.,0.,-1.)) ;
#37304=DIRECTION('',(0.,0.,-1.)) ;
#37305=DIRECTION('center_axis',(1.,0.,0.)) ;
#37306=DIRECTION('ref_axis',(0.,0.,-1.)) ;
#37307=DIRECTION('',(0.,0.,-1.)) ;
#37308=DIRECTION('center_axis',(0.,-1.,0.)) ;
#37309=DIRECTION('ref_axis',(0.,0.,-1.)) ;
#37310=DIRECTION('',(0.,0.,-1.)) ;
#37311=DIRECTION('center_axis',(-1.,0.,0.)) ;
#37312=DIRECTION('ref_axis',(0.,0.,1.)) ;
#46211=CARTESIAN_POINT('',(0.,0.,0.)) ;
#46212=CARTESIAN_POINT('Origin',(31.9,0.,44.)) ;
#46213=CARTESIAN_POINT('',(31.64,-3.18408167778312E-17,43.8)) ;
#46214=CARTESIAN_POINT('Origin',(31.9,0.,43.8)) ;
#46215=CARTESIAN_POINT('',(31.64,3.18408167778312E-17,44.2)) ;
#46216=CARTESIAN_POINT('',(31.64,-3.18408167778312E-17,44.)) ;
#46217=CARTESIAN_POINT('Origin',(31.9,0.,44.2)) ;
#46218=CARTESIAN_POINT('Origin',(32.1,0.,43.8)) ;
#46219=CARTESIAN_POINT('',(32.6,-1.,43.8)) ;
#46220=CARTESIAN_POINT('',(32.6,1.,43.8)) ;
#46221=CARTESIAN_POINT('',(32.6,0.,43.8)) ;
#46222=CARTESIAN_POINT('',(31.,-1.,43.8)) ;
#46223=CARTESIAN_POINT('',(32.1,-1.,43.8)) ;
#46224=CARTESIAN_POINT('',(31.,1.,43.8)) ;
#46225=CARTESIAN_POINT('',(31.,0.,43.8)) ;
#46226=CARTESIAN_POINT('',(32.1,1.,43.8)) ;
#46227=CARTESIAN_POINT('Origin',(31.,0.,44.)) ;
#46228=CARTESIAN_POINT('',(31.,1.,44.2)) ;
#46229=CARTESIAN_POINT('',(31.,1.,44.)) ;
#46230=CARTESIAN_POINT('',(31.,-1.,44.2)) ;
#46231=CARTESIAN_POINT('',(31.,-1.,44.)) ;
#46232=CARTESIAN_POINT('',(31.,0.,44.2)) ;
#46233=CARTESIAN_POINT('Origin',(32.9,1.,43.3)) ;
#46234=CARTESIAN_POINT('',(33.2,1.,44.2)) ;
#46235=CARTESIAN_POINT('',(33.2,1.,42.4)) ;
#46236=CARTESIAN_POINT('',(33.2,1.,43.3)) ;
#46237=CARTESIAN_POINT('',(32.6,1.,42.4)) ;
#46238=CARTESIAN_POINT('',(19.95,1.,42.4)) ;
#46239=CARTESIAN_POINT('',(32.6,1.,43.3)) ;
#46240=CARTESIAN_POINT('',(32.9,1.,44.2)) ;
#46241=CARTESIAN_POINT('Origin',(33.2,0.,43.3)) ;
#46242=CARTESIAN_POINT('',(33.2,-1.,44.2)) ;
#46243=CARTESIAN_POINT('',(33.2,-1.,42.4)) ;
#46244=CARTESIAN_POINT('',(33.2,-1.,43.3)) ;
#46245=CARTESIAN_POINT('',(33.2,0.,42.4)) ;
#46246=CARTESIAN_POINT('',(33.2,0.,44.2)) ;
#46247=CARTESIAN_POINT('Origin',(32.9,0.,44.2)) ;
#46248=CARTESIAN_POINT('',(32.9,-1.,44.2)) ;
#46249=CARTESIAN_POINT('Origin',(32.9,-1.,43.3)) ;
#46250=CARTESIAN_POINT('',(32.6,-1.,42.4)) ;
#46251=CARTESIAN_POINT('',(32.6,-1.,43.3)) ;
#46252=CARTESIAN_POINT('',(19.95,-1.,42.4)) ;
#46253=CARTESIAN_POINT('Origin',(32.6,0.,43.3)) ;
#46254=CARTESIAN_POINT('',(32.6,0.,42.4)) ;
#46255=CARTESIAN_POINT('Origin',(-17.5,0.,43.6)) ;
#46256=CARTESIAN_POINT('',(-18.,-5.02105187650415E-17,44.01)) ;
#46257=CARTESIAN_POINT('Origin',(-18.,0.,43.6)) ;
#46258=CARTESIAN_POINT('',(-17.,5.02105187650415E-17,44.01)) ;
#46259=CARTESIAN_POINT('',(-17.5,-5.02105187650415E-17,44.01)) ;
#46260=CARTESIAN_POINT('Origin',(-17.,0.,43.6)) ;
#46261=CARTESIAN_POINT('Origin',(-17.5,0.,44.6)) ;
#46262=CARTESIAN_POINT('',(-17.,-1.,44.6)) ;
#46263=CARTESIAN_POINT('',(-17.,1.,44.6)) ;
#46264=CARTESIAN_POINT('',(-17.,0.,44.6)) ;
#46265=CARTESIAN_POINT('',(-18.,1.,44.6)) ;
#46266=CARTESIAN_POINT('',(-17.5,1.,44.6)) ;
#46267=CARTESIAN_POINT('',(-18.,-1.,44.6)) ;
#46268=CARTESIAN_POINT('',(-18.,0.,44.6)) ;
#46269=CARTESIAN_POINT('',(-17.5,-1.,44.6)) ;
#46270=CARTESIAN_POINT('Origin',(-17.5,-1.,43.5)) ;
#46271=CARTESIAN_POINT('',(-18.,-1.,42.4)) ;
#46272=CARTESIAN_POINT('',(-18.,-1.,43.5)) ;
#46273=CARTESIAN_POINT('',(-17.,-1.,42.4)) ;
#46274=CARTESIAN_POINT('',(-5.25,-1.,42.4)) ;
#46275=CARTESIAN_POINT('',(-17.,-1.,43.5)) ;
#46276=CARTESIAN_POINT('Origin',(-18.,0.,43.5)) ;
#46277=CARTESIAN_POINT('',(-18.,1.,42.4)) ;
#46278=CARTESIAN_POINT('',(-18.,1.,43.5)) ;
#46279=CARTESIAN_POINT('',(-18.,0.,42.4)) ;
#46280=CARTESIAN_POINT('Origin',(-17.5,1.,43.5)) ;
#46281=CARTESIAN_POINT('',(-17.,1.,42.4)) ;
#46282=CARTESIAN_POINT('',(-17.,1.,43.5)) ;
#46283=CARTESIAN_POINT('',(-5.25,1.,42.4)) ;
#46284=CARTESIAN_POINT('Origin',(-17.,0.,43.5)) ;
#46285=CARTESIAN_POINT('',(-17.,0.,42.4)) ;
#46286=CARTESIAN_POINT('Origin',(-11.,-10.,42.4)) ;
#46287=CARTESIAN_POINT('',(-11.425,-10.,42.)) ;
#46288=CARTESIAN_POINT('Origin',(-11.,-10.,42.)) ;
#46289=CARTESIAN_POINT('',(-11.425,-10.,42.8)) ;
#46290=CARTESIAN_POINT('',(-11.425,-10.,42.4)) ;
#46291=CARTESIAN_POINT('Origin',(-11.,-10.,42.8)) ;
#46292=CARTESIAN_POINT('Origin',(-11.,10.,42.4)) ;
#46293=CARTESIAN_POINT('',(-11.425,10.,42.)) ;
#46294=CARTESIAN_POINT('Origin',(-11.,10.,42.)) ;
#46295=CARTESIAN_POINT('',(-11.425,10.,42.8)) ;
#46296=CARTESIAN_POINT('',(-11.425,10.,42.4)) ;
#46297=CARTESIAN_POINT('Origin',(-11.,10.,42.8)) ;
#46298=CARTESIAN_POINT('Origin',(11.,-10.,42.4)) ;
#46299=CARTESIAN_POINT('',(10.575,-10.,42.)) ;
#46300=CARTESIAN_POINT('Origin',(11.,-10.,42.)) ;
#46301=CARTESIAN_POINT('',(10.575,-10.,42.8)) ;
#46302=CARTESIAN_POINT('',(10.575,-10.,42.4)) ;
#46303=CARTESIAN_POINT('Origin',(11.,-10.,42.8)) ;
#46304=CARTESIAN_POINT('Origin',(11.,10.,42.4)) ;
#46305=CARTESIAN_POINT('',(10.575,10.,42.)) ;
#46306=CARTESIAN_POINT('Origin',(11.,10.,42.)) ;
#46307=CARTESIAN_POINT('',(10.575,10.,42.8)) ;
#46308=CARTESIAN_POINT('',(10.575,10.,42.4)) ;
#46309=CARTESIAN_POINT('Origin',(11.,10.,42.8)) ;
#46310=CARTESIAN_POINT('Origin',(7.,7.,42.4)) ;
#46311=CARTESIAN_POINT('',(5.95,7.,42.)) ;
#46312=CARTESIAN_POINT('Origin',(7.,7.,42.)) ;
#46313=CARTESIAN_POINT('',(5.95,7.,42.4)) ;
#46314=CARTESIAN_POINT('',(5.95,7.,42.4)) ;
#46315=CARTESIAN_POINT('',(8.03077640640442,7.2,42.4)) ;
#46316=CARTESIAN_POINT('Origin',(7.,7.,42.4)) ;
#46317=CARTESIAN_POINT('',(8.03077640640442,7.2,42.8)) ;
#46318=CARTESIAN_POINT('',(8.03077640640442,7.2,42.4)) ;
#46319=CARTESIAN_POINT('',(5.96922359359558,7.2,42.8)) ;
#46320=CARTESIAN_POINT('Origin',(7.,7.,42.8)) ;
#46321=CARTESIAN_POINT('',(5.96922359359558,7.2,42.4)) ;
#46322=CARTESIAN_POINT('',(5.96922359359558,7.2,42.4)) ;
#46323=CARTESIAN_POINT('Origin',(7.,7.,42.4)) ;
#46324=CARTESIAN_POINT('Origin',(7.,0.,42.4)) ;
#46325=CARTESIAN_POINT('',(-16.,7.2,42.4)) ;
#46326=CARTESIAN_POINT('',(3.5,7.2,42.4)) ;
#46327=CARTESIAN_POINT('',(-16.,12.,42.4)) ;
#46328=CARTESIAN_POINT('',(-16.,4.8,42.4)) ;
#46329=CARTESIAN_POINT('',(-20.,12.,42.4)) ;
#46330=CARTESIAN_POINT('',(7.,12.,42.4)) ;
#46331=CARTESIAN_POINT('',(-20.,-12.,42.4)) ;
#46332=CARTESIAN_POINT('',(-20.,0.,42.4)) ;
#46333=CARTESIAN_POINT('',(-16.,-12.,42.4)) ;
#46334=CARTESIAN_POINT('',(7.,-12.,42.4)) ;
#46335=CARTESIAN_POINT('',(-16.,-7.2,42.4)) ;
#46336=CARTESIAN_POINT('',(-16.,-4.8,42.4)) ;
#46337=CARTESIAN_POINT('',(-2.19374109684803,-7.2,42.4)) ;
#46338=CARTESIAN_POINT('',(3.5,-7.2,42.4)) ;
#46339=CARTESIAN_POINT('',(-1.37550241686044,-6.35279411764706,42.4)) ;
#46340=CARTESIAN_POINT('Origin',(0.,-8.5,42.4)) ;
#46341=CARTESIAN_POINT('',(1.37550241686044,-6.35279411764706,42.4)) ;
#46342=CARTESIAN_POINT('Origin',(0.,0.,42.4)) ;
#46343=CARTESIAN_POINT('',(2.19374109684803,-7.2,42.4)) ;
#46344=CARTESIAN_POINT('Origin',(0.,-8.5,42.4)) ;
#46345=CARTESIAN_POINT('',(16.,-7.2,42.4)) ;
#46346=CARTESIAN_POINT('',(3.5,-7.2,42.4)) ;
#46347=CARTESIAN_POINT('',(16.,-12.,42.4)) ;
#46348=CARTESIAN_POINT('',(16.,-4.8,42.4)) ;
#46349=CARTESIAN_POINT('',(34.,-12.,42.4)) ;
#46350=CARTESIAN_POINT('',(7.,-12.,42.4)) ;
#46351=CARTESIAN_POINT('',(34.,12.,42.4)) ;
#46352=CARTESIAN_POINT('',(34.,0.,42.4)) ;
#46353=CARTESIAN_POINT('',(16.,12.,42.4)) ;
#46354=CARTESIAN_POINT('',(7.,12.,42.4)) ;
#46355=CARTESIAN_POINT('',(16.,7.2,42.4)) ;
#46356=CARTESIAN_POINT('',(16.,4.8,42.4)) ;
#46357=CARTESIAN_POINT('',(3.5,7.2,42.4)) ;
#46358=CARTESIAN_POINT('Origin',(0.,7.2,42.6)) ;
#46359=CARTESIAN_POINT('',(-16.,7.2,42.8)) ;
#46360=CARTESIAN_POINT('',(0.,7.2,42.8)) ;
#46361=CARTESIAN_POINT('',(-16.,7.2,42.6)) ;
#46362=CARTESIAN_POINT('Origin',(0.,-9.6,42.8)) ;
#46363=CARTESIAN_POINT('',(2.19374109684803,-7.2,42.8)) ;
#46364=CARTESIAN_POINT('',(-2.19374109684803,-7.2,42.8)) ;
#46365=CARTESIAN_POINT('Origin',(0.,-8.5,42.8)) ;
#46366=CARTESIAN_POINT('',(-16.,-7.2,42.8)) ;
#46367=CARTESIAN_POINT('',(0.,-7.2,42.8)) ;
#46368=CARTESIAN_POINT('',(-16.,-12.,42.8)) ;
#46369=CARTESIAN_POINT('',(-16.,-9.6,42.8)) ;
#46370=CARTESIAN_POINT('',(16.,-12.,42.8)) ;
#46371=CARTESIAN_POINT('',(0.,-12.,42.8)) ;
#46372=CARTESIAN_POINT('',(16.,-7.2,42.8)) ;
#46373=CARTESIAN_POINT('',(16.,-9.6,42.8)) ;
#46374=CARTESIAN_POINT('',(0.,-7.2,42.8)) ;
#46375=CARTESIAN_POINT('Origin',(0.,-7.2,42.6)) ;
#46376=CARTESIAN_POINT('',(-2.19374109684803,-7.2,42.4)) ;
#46377=CARTESIAN_POINT('',(-16.,-7.2,42.6)) ;
#46378=CARTESIAN_POINT('Origin',(-16.,-9.6,42.6)) ;
#46379=CARTESIAN_POINT('',(-16.,-12.,42.6)) ;
#46380=CARTESIAN_POINT('Origin',(0.,-7.2,42.6)) ;
#46381=CARTESIAN_POINT('',(2.19374109684803,-7.2,42.4)) ;
#46382=CARTESIAN_POINT('',(16.,-7.2,42.6)) ;
#46383=CARTESIAN_POINT('Origin',(16.,-9.6,42.6)) ;
#46384=CARTESIAN_POINT('',(16.,-12.,42.6)) ;
#46385=CARTESIAN_POINT('Origin',(0.,9.6,42.8)) ;
#46386=CARTESIAN_POINT('',(16.,7.2,42.8)) ;
#46387=CARTESIAN_POINT('',(0.,7.2,42.8)) ;
#46388=CARTESIAN_POINT('',(16.,12.,42.8)) ;
#46389=CARTESIAN_POINT('',(16.,9.6,42.8)) ;
#46390=CARTESIAN_POINT('',(-16.,12.,42.8)) ;
#46391=CARTESIAN_POINT('',(0.,12.,42.8)) ;
#46392=CARTESIAN_POINT('',(-16.,9.6,42.8)) ;
#46393=CARTESIAN_POINT('Origin',(0.,7.2,42.6)) ;
#46394=CARTESIAN_POINT('',(16.,7.2,42.6)) ;
#46395=CARTESIAN_POINT('Origin',(-16.,9.6,42.6)) ;
#46396=CARTESIAN_POINT('',(-16.,12.,42.6)) ;
#46397=CARTESIAN_POINT('Origin',(16.,9.6,42.6)) ;
#46398=CARTESIAN_POINT('',(16.,12.,42.6)) ;
#46399=CARTESIAN_POINT('Origin',(0.,-8.5,42.2)) ;
#46400=CARTESIAN_POINT('',(1.37550241686044,-6.35279411764706,42.)) ;
#46401=CARTESIAN_POINT('',(1.37550241686045,-6.35279411764706,42.2)) ;
#46402=CARTESIAN_POINT('',(-1.37550241686044,-6.35279411764706,42.)) ;
#46403=CARTESIAN_POINT('Origin',(0.,-8.5,42.)) ;
#46404=CARTESIAN_POINT('',(-1.37550241686045,-6.35279411764706,42.2)) ;
#46405=CARTESIAN_POINT('Origin',(7.,0.,42.)) ;
#46406=CARTESIAN_POINT('',(34.,12.,42.)) ;
#46407=CARTESIAN_POINT('',(34.,-12.,42.)) ;
#46408=CARTESIAN_POINT('',(34.,0.,42.)) ;
#46409=CARTESIAN_POINT('',(-20.,-12.,42.)) ;
#46410=CARTESIAN_POINT('',(7.,-12.,42.)) ;
#46411=CARTESIAN_POINT('',(-20.,12.,42.)) ;
#46412=CARTESIAN_POINT('',(-20.,0.,42.)) ;
#46413=CARTESIAN_POINT('',(7.,12.,42.)) ;
#46414=CARTESIAN_POINT('Origin',(0.,0.,42.)) ;
#46415=CARTESIAN_POINT('Origin',(0.,0.,42.2)) ;
#46416=CARTESIAN_POINT('Origin',(7.,-12.,42.2)) ;
#46417=CARTESIAN_POINT('',(-20.,-12.,42.2)) ;
#46418=CARTESIAN_POINT('',(34.,-12.,42.2)) ;
#46419=CARTESIAN_POINT('Origin',(-20.,0.,42.2)) ;
#46420=CARTESIAN_POINT('',(-20.,12.,42.2)) ;
#46421=CARTESIAN_POINT('Origin',(7.,12.,42.2)) ;
#46422=CARTESIAN_POINT('',(34.,12.,42.2)) ;
#46423=CARTESIAN_POINT('Origin',(34.,0.,42.2)) ;
#50359=UNCERTAINTY_MEASURE_WITH_UNIT(LENGTH_MEASURE(0.001),#50441,
'DISTANCE_ACCURACY_VALUE',
'Maximum model space distance between geometric entities at asserted c
onnectivities') ;
#50387=UNCERTAINTY_MEASURE_WITH_UNIT(LENGTH_MEASURE(0.001),#50441,
'DISTANCE_ACCURACY_VALUE',
'Maximum model space distance between geometric entities at asserted c
onnectivities') ;
#50412=(
GEOMETRIC_REPRESENTATION_CONTEXT(3)
GLOBAL_UNCERTAINTY_ASSIGNED_CONTEXT((#50359))
GLOBAL_UNIT_ASSIGNED_CONTEXT((#50441,#50443,#50444))
REPRESENTATION_CONTEXT('','3D')
) ;
#50440=(
GEOMETRIC_REPRESENTATION_CONTEXT(3)
GLOBAL_UNCERTAINTY_ASSIGNED_CONTEXT((#50387))
GLOBAL_UNIT_ASSIGNED_CONTEXT((#50441,#50443,#50444))
REPRESENTATION_CONTEXT('','3D')
) ;
#50441=(
LENGTH_UNIT()
NAMED_UNIT(*)
SI_UNIT(.CENTI.,.METRE.)
) ;
#50443=(
NAMED_UNIT(*)
PLANE_ANGLE_UNIT()
SI_UNIT($,.RADIAN.)
) ;
#50444=(
NAMED_UNIT(*)
SI_UNIT($,.STERADIAN.)
SOLID_ANGLE_UNIT()
) ;
#50469=SHAPE_DEFINITION_REPRESENTATION(#50545,#50643) ;
#50545=PRODUCT_DEFINITION_SHAPE('',$,#50696) ;
#50643=SHAPE_REPRESENTATION('',(#30674),#50412) ;
#50671=PRODUCT_DEFINITION_CONTEXT('part definition',#50829,'design') ;
#50696=PRODUCT_DEFINITION('GATE_HOUSING_PLATE',
'GATE_HOUSING_PLATE',#50748,#50671) ;
#50748=PRODUCT_DEFINITION_FORMATION('',$,#50855) ;
#50829=APPLICATION_CONTEXT(
'Core Data for Automotive Mechanical Design Process') ;
#50830=PRODUCT_CONTEXT('part definition',#50829,'mechanical') ;
#50855=PRODUCT('GATE_HOUSING_PLATE','GATE_HOUSING_PLATE',$,(#50830)) ;
#50885=PRESENTATION_STYLE_ASSIGNMENT((#50892)) ;
#50892=SURFACE_STYLE_USAGE(.BOTH.,#50899) ;
#50899=SURFACE_SIDE_STYLE('',(#50906)) ;
#50906=SURFACE_STYLE_FILL_AREA(#50913) ;
#50913=FILL_AREA_STYLE('Steel - Galvanized (Small)',(#50920)) ;
#50920=FILL_AREA_STYLE_COLOUR('Steel - Galvanized (Small)',#50927) ;
#50927=COLOUR_RGB('Steel - Galvanized (Small)', 0.09019608, 0.27058824, 0.51372549) ;
ENDSEC;
END-ISO-10303-21;
